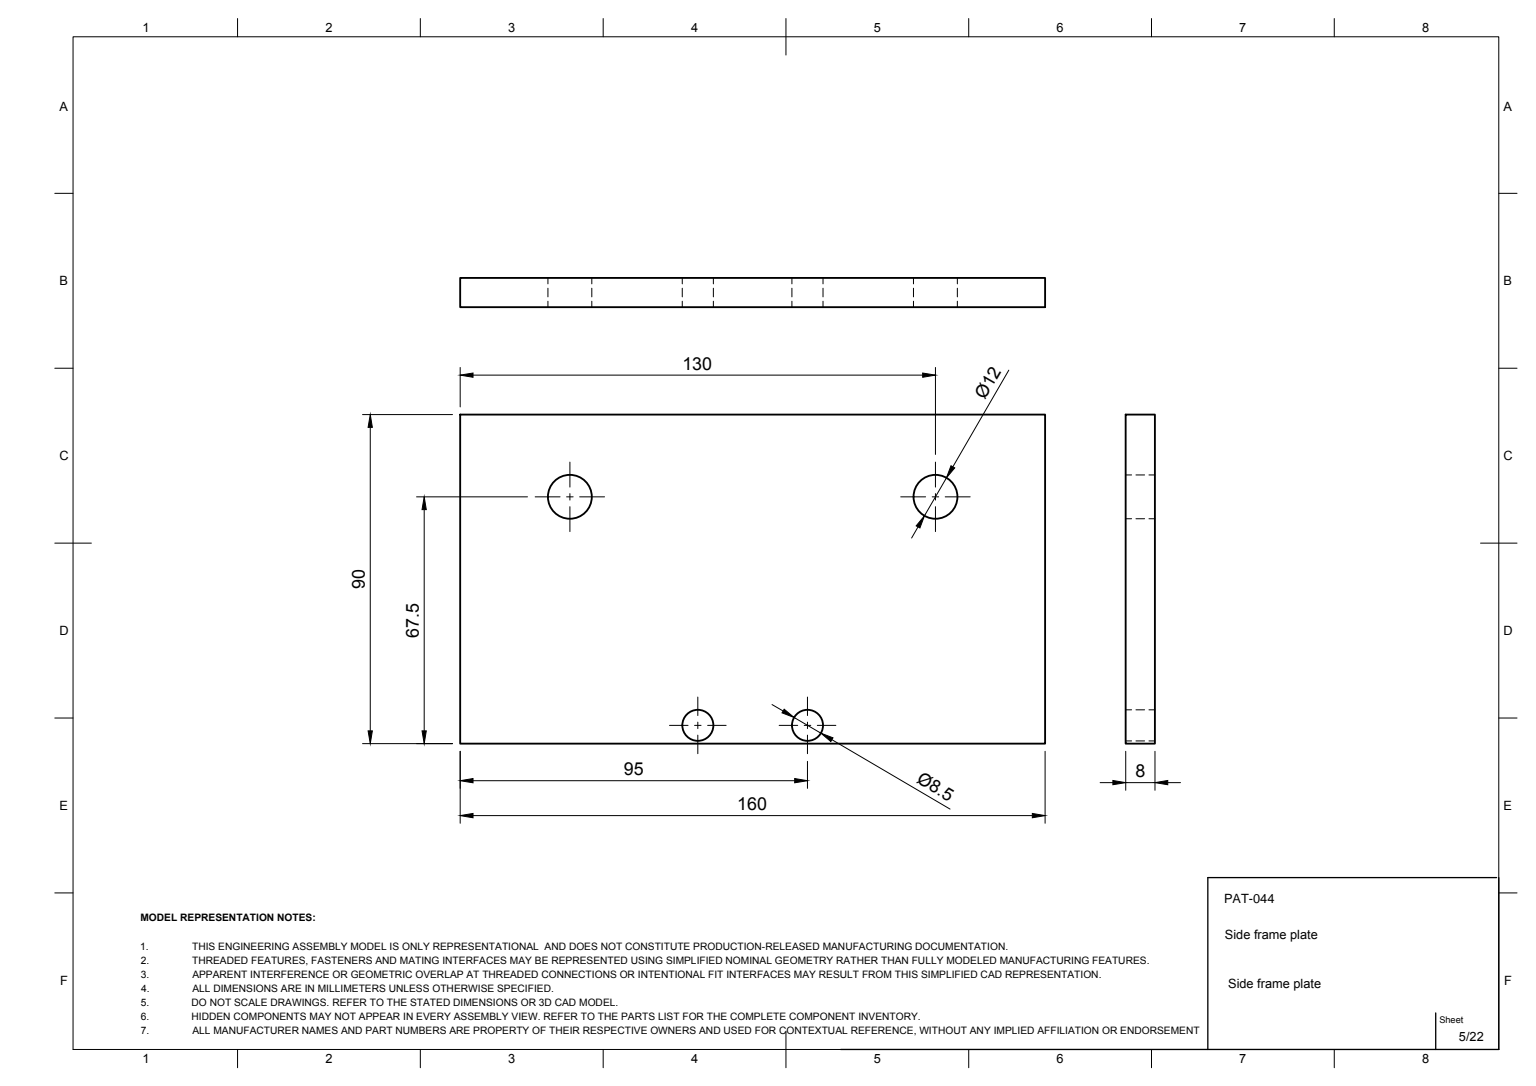
ISO-10303-21;
HEADER;
/* Generated by software containing ST-Developer
 * from STEP Tools, Inc. (www.steptools.com) 
 */

FILE_DESCRIPTION(
/* description */ ('Four-wheel beam trolley'),
/* implementation_level */ '2;1');

FILE_NAME(
/* name */ 'Side frame plate.step',
/* time_stamp */ '2026-10-29T16:22:06-07:00',
/* author */ (''),
/* organization */ (''),
/* preprocessor_version */ 'ST-DEVELOPER v20.2',
/* originating_system */ 'Autodesk Translation Framework v15.17.0.0',
/* authorisation */ '');

FILE_SCHEMA (('AUTOMOTIVE_DESIGN { 1 0 10303 214 3 1 1 }'));
ENDSEC;

DATA;
#10=MECHANICAL_DESIGN_GEOMETRIC_PRESENTATION_REPRESENTATION('',(#279),#4777);
#245=SHAPE_REPRESENTATION_RELATIONSHIP('SRR','None',#4874,#262);
#262=ADVANCED_BREP_SHAPE_REPRESENTATION('',(#303),#4759);
#279=STYLED_ITEM('',(#5035),#303);
#303=MANIFOLD_SOLID_BREP('Body1',#2366);
#328=FACE_BOUND('',#612,.T.);
#329=FACE_BOUND('',#613,.T.);
#330=FACE_BOUND('',#614,.T.);
#331=FACE_BOUND('',#615,.T.);
#332=FACE_BOUND('',#618,.T.);
#333=FACE_BOUND('',#619,.T.);
#334=FACE_BOUND('',#620,.T.);
#335=FACE_BOUND('',#621,.T.);
#375=PLANE('',#2617);
#376=PLANE('',#2618);
#377=PLANE('',#2619);
#378=PLANE('',#2620);
#379=PLANE('',#2621);
#380=PLANE('',#2622);
#456=FACE_OUTER_BOUND('',#607,.T.);
#457=FACE_OUTER_BOUND('',#608,.T.);
#458=FACE_OUTER_BOUND('',#609,.T.);
#459=FACE_OUTER_BOUND('',#610,.T.);
#460=FACE_OUTER_BOUND('',#611,.T.);
#461=FACE_OUTER_BOUND('',#616,.T.);
#462=FACE_OUTER_BOUND('',#617,.T.);
#463=FACE_OUTER_BOUND('',#622,.T.);
#464=FACE_OUTER_BOUND('',#623,.T.);
#465=FACE_OUTER_BOUND('',#624,.T.);
#607=EDGE_LOOP('',(#1673,#1674,#1675,#1676));
#608=EDGE_LOOP('',(#1677,#1678,#1679,#1680));
#609=EDGE_LOOP('',(#1681,#1682,#1683,#1684));
#610=EDGE_LOOP('',(#1685,#1686,#1687,#1688));
#611=EDGE_LOOP('',(#1689,#1690,#1691,#1692));
#612=EDGE_LOOP('',(#1693));
#613=EDGE_LOOP('',(#1694));
#614=EDGE_LOOP('',(#1695));
#615=EDGE_LOOP('',(#1696));
#616=EDGE_LOOP('',(#1697,#1698,#1699,#1700));
#617=EDGE_LOOP('',(#1701,#1702,#1703,#1704));
#618=EDGE_LOOP('',(#1705));
#619=EDGE_LOOP('',(#1706));
#620=EDGE_LOOP('',(#1707));
#621=EDGE_LOOP('',(#1708));
#622=EDGE_LOOP('',(#1709,#1710,#1711,#1712));
#623=EDGE_LOOP('',(#1713,#1714,#1715,#1716));
#624=EDGE_LOOP('',(#1717,#1718,#1719,#1720));
#793=LINE('',#3823,#916);
#794=LINE('',#3829,#917);
#795=LINE('',#3835,#918);
#796=LINE('',#3841,#919);
#797=LINE('',#3846,#920);
#798=LINE('',#3848,#921);
#799=LINE('',#3850,#922);
#800=LINE('',#3851,#923);
#801=LINE('',#3854,#924);
#802=LINE('',#3856,#925);
#803=LINE('',#3857,#926);
#804=LINE('',#3860,#927);
#805=LINE('',#3862,#928);
#806=LINE('',#3863,#929);
#807=LINE('',#3865,#930);
#808=LINE('',#3866,#931);
#916=VECTOR('',#3004,0.425);
#917=VECTOR('',#3011,0.425);
#918=VECTOR('',#3018,0.6);
#919=VECTOR('',#3025,0.6);
#920=VECTOR('',#3030,1.);
#921=VECTOR('',#3031,1.);
#922=VECTOR('',#3032,1.);
#923=VECTOR('',#3033,1.);
#924=VECTOR('',#3036,1.);
#925=VECTOR('',#3037,1.);
#926=VECTOR('',#3038,1.);
#927=VECTOR('',#3041,1.);
#928=VECTOR('',#3042,1.);
#929=VECTOR('',#3043,1.);
#930=VECTOR('',#3046,1.);
#931=VECTOR('',#3047,1.);
#1031=CIRCLE('',#2606,0.425);
#1032=CIRCLE('',#2607,0.425);
#1033=CIRCLE('',#2609,0.425);
#1034=CIRCLE('',#2610,0.425);
#1035=CIRCLE('',#2612,0.6);
#1036=CIRCLE('',#2613,0.6);
#1037=CIRCLE('',#2615,0.6);
#1038=CIRCLE('',#2616,0.6);
#1177=VERTEX_POINT('',#3820);
#1178=VERTEX_POINT('',#3822);
#1179=VERTEX_POINT('',#3826);
#1180=VERTEX_POINT('',#3828);
#1181=VERTEX_POINT('',#3832);
#1182=VERTEX_POINT('',#3834);
#1183=VERTEX_POINT('',#3838);
#1184=VERTEX_POINT('',#3840);
#1185=VERTEX_POINT('',#3844);
#1186=VERTEX_POINT('',#3845);
#1187=VERTEX_POINT('',#3847);
#1188=VERTEX_POINT('',#3849);
#1189=VERTEX_POINT('',#3853);
#1190=VERTEX_POINT('',#3855);
#1191=VERTEX_POINT('',#3859);
#1192=VERTEX_POINT('',#3861);
#1374=EDGE_CURVE('',#1177,#1177,#1031,.T.);
#1375=EDGE_CURVE('',#1177,#1178,#793,.T.);
#1376=EDGE_CURVE('',#1178,#1178,#1032,.T.);
#1377=EDGE_CURVE('',#1179,#1179,#1033,.T.);
#1378=EDGE_CURVE('',#1179,#1180,#794,.T.);
#1379=EDGE_CURVE('',#1180,#1180,#1034,.T.);
#1380=EDGE_CURVE('',#1181,#1181,#1035,.T.);
#1381=EDGE_CURVE('',#1181,#1182,#795,.T.);
#1382=EDGE_CURVE('',#1182,#1182,#1036,.T.);
#1383=EDGE_CURVE('',#1183,#1183,#1037,.T.);
#1384=EDGE_CURVE('',#1183,#1184,#796,.T.);
#1385=EDGE_CURVE('',#1184,#1184,#1038,.T.);
#1386=EDGE_CURVE('',#1185,#1186,#797,.T.);
#1387=EDGE_CURVE('',#1186,#1187,#798,.T.);
#1388=EDGE_CURVE('',#1188,#1187,#799,.T.);
#1389=EDGE_CURVE('',#1185,#1188,#800,.T.);
#1390=EDGE_CURVE('',#1189,#1185,#801,.T.);
#1391=EDGE_CURVE('',#1190,#1188,#802,.T.);
#1392=EDGE_CURVE('',#1189,#1190,#803,.T.);
#1393=EDGE_CURVE('',#1191,#1189,#804,.T.);
#1394=EDGE_CURVE('',#1192,#1190,#805,.T.);
#1395=EDGE_CURVE('',#1191,#1192,#806,.T.);
#1396=EDGE_CURVE('',#1186,#1191,#807,.T.);
#1397=EDGE_CURVE('',#1187,#1192,#808,.T.);
#1673=ORIENTED_EDGE('',*,*,#1374,.F.);
#1674=ORIENTED_EDGE('',*,*,#1375,.T.);
#1675=ORIENTED_EDGE('',*,*,#1376,.F.);
#1676=ORIENTED_EDGE('',*,*,#1375,.F.);
#1677=ORIENTED_EDGE('',*,*,#1377,.F.);
#1678=ORIENTED_EDGE('',*,*,#1378,.T.);
#1679=ORIENTED_EDGE('',*,*,#1379,.F.);
#1680=ORIENTED_EDGE('',*,*,#1378,.F.);
#1681=ORIENTED_EDGE('',*,*,#1380,.F.);
#1682=ORIENTED_EDGE('',*,*,#1381,.T.);
#1683=ORIENTED_EDGE('',*,*,#1382,.F.);
#1684=ORIENTED_EDGE('',*,*,#1381,.F.);
#1685=ORIENTED_EDGE('',*,*,#1383,.F.);
#1686=ORIENTED_EDGE('',*,*,#1384,.T.);
#1687=ORIENTED_EDGE('',*,*,#1385,.F.);
#1688=ORIENTED_EDGE('',*,*,#1384,.F.);
#1689=ORIENTED_EDGE('',*,*,#1386,.T.);
#1690=ORIENTED_EDGE('',*,*,#1387,.T.);
#1691=ORIENTED_EDGE('',*,*,#1388,.F.);
#1692=ORIENTED_EDGE('',*,*,#1389,.F.);
#1693=ORIENTED_EDGE('',*,*,#1376,.T.);
#1694=ORIENTED_EDGE('',*,*,#1379,.T.);
#1695=ORIENTED_EDGE('',*,*,#1382,.T.);
#1696=ORIENTED_EDGE('',*,*,#1385,.T.);
#1697=ORIENTED_EDGE('',*,*,#1390,.T.);
#1698=ORIENTED_EDGE('',*,*,#1389,.T.);
#1699=ORIENTED_EDGE('',*,*,#1391,.F.);
#1700=ORIENTED_EDGE('',*,*,#1392,.F.);
#1701=ORIENTED_EDGE('',*,*,#1393,.T.);
#1702=ORIENTED_EDGE('',*,*,#1392,.T.);
#1703=ORIENTED_EDGE('',*,*,#1394,.F.);
#1704=ORIENTED_EDGE('',*,*,#1395,.F.);
#1705=ORIENTED_EDGE('',*,*,#1374,.T.);
#1706=ORIENTED_EDGE('',*,*,#1377,.T.);
#1707=ORIENTED_EDGE('',*,*,#1380,.T.);
#1708=ORIENTED_EDGE('',*,*,#1383,.T.);
#1709=ORIENTED_EDGE('',*,*,#1396,.T.);
#1710=ORIENTED_EDGE('',*,*,#1395,.T.);
#1711=ORIENTED_EDGE('',*,*,#1397,.F.);
#1712=ORIENTED_EDGE('',*,*,#1387,.F.);
#1713=ORIENTED_EDGE('',*,*,#1397,.T.);
#1714=ORIENTED_EDGE('',*,*,#1394,.T.);
#1715=ORIENTED_EDGE('',*,*,#1391,.T.);
#1716=ORIENTED_EDGE('',*,*,#1388,.T.);
#1717=ORIENTED_EDGE('',*,*,#1396,.F.);
#1718=ORIENTED_EDGE('',*,*,#1386,.F.);
#1719=ORIENTED_EDGE('',*,*,#1390,.F.);
#1720=ORIENTED_EDGE('',*,*,#1393,.F.);
#2179=CYLINDRICAL_SURFACE('',#2605,0.425);
#2180=CYLINDRICAL_SURFACE('',#2608,0.425);
#2181=CYLINDRICAL_SURFACE('',#2611,0.6);
#2182=CYLINDRICAL_SURFACE('',#2614,0.6);
#2232=ADVANCED_FACE('',(#456),#2179,.F.);
#2233=ADVANCED_FACE('',(#457),#2180,.F.);
#2234=ADVANCED_FACE('',(#458),#2181,.F.);
#2235=ADVANCED_FACE('',(#459),#2182,.F.);
#2236=ADVANCED_FACE('',(#460,#328,#329,#330,#331),#375,.T.);
#2237=ADVANCED_FACE('',(#461),#376,.T.);
#2238=ADVANCED_FACE('',(#462,#332,#333,#334,#335),#377,.T.);
#2239=ADVANCED_FACE('',(#463),#378,.T.);
#2240=ADVANCED_FACE('',(#464),#379,.T.);
#2241=ADVANCED_FACE('',(#465),#380,.F.);
#2366=CLOSED_SHELL('',(#2232,#2233,#2234,#2235,#2236,#2237,#2238,#2239,
#2240,#2241));
#2604=AXIS2_PLACEMENT_3D('',#3818,#2998,#2999);
#2605=AXIS2_PLACEMENT_3D('',#3819,#3000,#3001);
#2606=AXIS2_PLACEMENT_3D('',#3821,#3002,#3003);
#2607=AXIS2_PLACEMENT_3D('',#3824,#3005,#3006);
#2608=AXIS2_PLACEMENT_3D('',#3825,#3007,#3008);
#2609=AXIS2_PLACEMENT_3D('',#3827,#3009,#3010);
#2610=AXIS2_PLACEMENT_3D('',#3830,#3012,#3013);
#2611=AXIS2_PLACEMENT_3D('',#3831,#3014,#3015);
#2612=AXIS2_PLACEMENT_3D('',#3833,#3016,#3017);
#2613=AXIS2_PLACEMENT_3D('',#3836,#3019,#3020);
#2614=AXIS2_PLACEMENT_3D('',#3837,#3021,#3022);
#2615=AXIS2_PLACEMENT_3D('',#3839,#3023,#3024);
#2616=AXIS2_PLACEMENT_3D('',#3842,#3026,#3027);
#2617=AXIS2_PLACEMENT_3D('',#3843,#3028,#3029);
#2618=AXIS2_PLACEMENT_3D('',#3852,#3034,#3035);
#2619=AXIS2_PLACEMENT_3D('',#3858,#3039,#3040);
#2620=AXIS2_PLACEMENT_3D('',#3864,#3044,#3045);
#2621=AXIS2_PLACEMENT_3D('',#3867,#3048,#3049);
#2622=AXIS2_PLACEMENT_3D('',#3868,#3050,#3051);
#2998=DIRECTION('axis',(0.,0.,1.));
#2999=DIRECTION('refdir',(1.,0.,0.));
#3000=DIRECTION('center_axis',(0.,1.,0.));
#3001=DIRECTION('ref_axis',(1.,0.,0.));
#3002=DIRECTION('center_axis',(0.,1.,0.));
#3003=DIRECTION('ref_axis',(1.,0.,0.));
#3004=DIRECTION('',(0.,1.,0.));
#3005=DIRECTION('center_axis',(0.,-1.,0.));
#3006=DIRECTION('ref_axis',(1.,0.,0.));
#3007=DIRECTION('center_axis',(0.,1.,0.));
#3008=DIRECTION('ref_axis',(1.,0.,0.));
#3009=DIRECTION('center_axis',(0.,1.,0.));
#3010=DIRECTION('ref_axis',(1.,0.,0.));
#3011=DIRECTION('',(0.,1.,0.));
#3012=DIRECTION('center_axis',(0.,-1.,0.));
#3013=DIRECTION('ref_axis',(1.,0.,0.));
#3014=DIRECTION('center_axis',(0.,1.,0.));
#3015=DIRECTION('ref_axis',(1.,0.,0.));
#3016=DIRECTION('center_axis',(0.,1.,0.));
#3017=DIRECTION('ref_axis',(1.,0.,0.));
#3018=DIRECTION('',(0.,1.,0.));
#3019=DIRECTION('center_axis',(0.,-1.,0.));
#3020=DIRECTION('ref_axis',(1.,0.,0.));
#3021=DIRECTION('center_axis',(0.,1.,0.));
#3022=DIRECTION('ref_axis',(1.,0.,0.));
#3023=DIRECTION('center_axis',(0.,1.,0.));
#3024=DIRECTION('ref_axis',(1.,0.,0.));
#3025=DIRECTION('',(0.,1.,0.));
#3026=DIRECTION('center_axis',(0.,-1.,0.));
#3027=DIRECTION('ref_axis',(1.,0.,0.));
#3028=DIRECTION('center_axis',(0.,1.,0.));
#3029=DIRECTION('ref_axis',(-1.,0.,0.));
#3030=DIRECTION('',(-1.,0.,0.));
#3031=DIRECTION('',(0.,0.,1.));
#3032=DIRECTION('',(-1.,0.,0.));
#3033=DIRECTION('',(0.,0.,1.));
#3034=DIRECTION('center_axis',(1.,0.,0.));
#3035=DIRECTION('ref_axis',(0.,1.,0.));
#3036=DIRECTION('',(0.,1.,0.));
#3037=DIRECTION('',(0.,1.,0.));
#3038=DIRECTION('',(0.,0.,1.));
#3039=DIRECTION('center_axis',(0.,-1.,0.));
#3040=DIRECTION('ref_axis',(1.,0.,0.));
#3041=DIRECTION('',(1.,0.,0.));
#3042=DIRECTION('',(1.,0.,0.));
#3043=DIRECTION('',(0.,0.,1.));
#3044=DIRECTION('center_axis',(-1.,0.,0.));
#3045=DIRECTION('ref_axis',(0.,-1.,0.));
#3046=DIRECTION('',(0.,-1.,0.));
#3047=DIRECTION('',(0.,-1.,0.));
#3048=DIRECTION('center_axis',(0.,0.,1.));
#3049=DIRECTION('ref_axis',(1.,0.,0.));
#3050=DIRECTION('center_axis',(0.,0.,1.));
#3051=DIRECTION('ref_axis',(1.,0.,0.));
#3818=CARTESIAN_POINT('',(0.,0.,0.));
#3819=CARTESIAN_POINT('Origin',(-1.5,5.4,7.5));
#3820=CARTESIAN_POINT('',(-1.925,5.5,7.5));
#3821=CARTESIAN_POINT('Origin',(-1.5,5.5,7.5));
#3822=CARTESIAN_POINT('',(-1.925,6.3,7.5));
#3823=CARTESIAN_POINT('',(-1.925,5.4,7.5));
#3824=CARTESIAN_POINT('Origin',(-1.5,6.3,7.5));
#3825=CARTESIAN_POINT('Origin',(1.5,5.4,7.5));
#3826=CARTESIAN_POINT('',(1.075,5.5,7.5));
#3827=CARTESIAN_POINT('Origin',(1.5,5.5,7.5));
#3828=CARTESIAN_POINT('',(1.075,6.3,7.5));
#3829=CARTESIAN_POINT('',(1.075,5.4,7.5));
#3830=CARTESIAN_POINT('Origin',(1.5,6.3,7.5));
#3831=CARTESIAN_POINT('Origin',(-5.,5.4,13.75));
#3832=CARTESIAN_POINT('',(-5.6,5.5,13.75));
#3833=CARTESIAN_POINT('Origin',(-5.,5.5,13.75));
#3834=CARTESIAN_POINT('',(-5.6,6.3,13.75));
#3835=CARTESIAN_POINT('',(-5.6,5.4,13.75));
#3836=CARTESIAN_POINT('Origin',(-5.,6.3,13.75));
#3837=CARTESIAN_POINT('Origin',(5.,5.4,13.75));
#3838=CARTESIAN_POINT('',(4.4,5.5,13.75));
#3839=CARTESIAN_POINT('Origin',(5.,5.5,13.75));
#3840=CARTESIAN_POINT('',(4.4,6.3,13.75));
#3841=CARTESIAN_POINT('',(4.4,5.4,13.75));
#3842=CARTESIAN_POINT('Origin',(5.,6.3,13.75));
#3843=CARTESIAN_POINT('Origin',(8.,6.3,7.));
#3844=CARTESIAN_POINT('',(8.,6.3,7.));
#3845=CARTESIAN_POINT('',(-8.,6.3,7.));
#3846=CARTESIAN_POINT('',(8.,6.3,7.));
#3847=CARTESIAN_POINT('',(-8.,6.3,16.));
#3848=CARTESIAN_POINT('',(-8.,6.3,7.));
#3849=CARTESIAN_POINT('',(8.,6.3,16.));
#3850=CARTESIAN_POINT('',(8.,6.3,16.));
#3851=CARTESIAN_POINT('',(8.,6.3,7.));
#3852=CARTESIAN_POINT('Origin',(8.,5.5,7.));
#3853=CARTESIAN_POINT('',(8.,5.5,7.));
#3854=CARTESIAN_POINT('',(8.,5.5,7.));
#3855=CARTESIAN_POINT('',(8.,5.5,16.));
#3856=CARTESIAN_POINT('',(8.,5.5,16.));
#3857=CARTESIAN_POINT('',(8.,5.5,7.));
#3858=CARTESIAN_POINT('Origin',(-8.,5.5,7.));
#3859=CARTESIAN_POINT('',(-8.,5.5,7.));
#3860=CARTESIAN_POINT('',(-8.,5.5,7.));
#3861=CARTESIAN_POINT('',(-8.,5.5,16.));
#3862=CARTESIAN_POINT('',(-8.,5.5,16.));
#3863=CARTESIAN_POINT('',(-8.,5.5,7.));
#3864=CARTESIAN_POINT('Origin',(-8.,6.3,7.));
#3865=CARTESIAN_POINT('',(-8.,6.3,7.));
#3866=CARTESIAN_POINT('',(-8.,6.3,16.));
#3867=CARTESIAN_POINT('Origin',(0.,5.9,16.));
#3868=CARTESIAN_POINT('Origin',(0.,5.9,7.));
#4737=UNCERTAINTY_MEASURE_WITH_UNIT(LENGTH_MEASURE(0.001),#4778,
'DISTANCE_ACCURACY_VALUE',
'Maximum model space distance between geometric entities at asserted c
onnectivities');
#4755=UNCERTAINTY_MEASURE_WITH_UNIT(LENGTH_MEASURE(0.001),#4778,
'DISTANCE_ACCURACY_VALUE',
'Maximum model space distance between geometric entities at asserted c
onnectivities');
#4759=(
GEOMETRIC_REPRESENTATION_CONTEXT(3)
GLOBAL_UNCERTAINTY_ASSIGNED_CONTEXT((#4737))
GLOBAL_UNIT_ASSIGNED_CONTEXT((#4778,#4780,#4781))
REPRESENTATION_CONTEXT('','3D')
);
#4777=(
GEOMETRIC_REPRESENTATION_CONTEXT(3)
GLOBAL_UNCERTAINTY_ASSIGNED_CONTEXT((#4755))
GLOBAL_UNIT_ASSIGNED_CONTEXT((#4778,#4780,#4781))
REPRESENTATION_CONTEXT('','3D')
);
#4778=(
LENGTH_UNIT()
NAMED_UNIT(*)
SI_UNIT(.CENTI.,.METRE.)
);
#4780=(
NAMED_UNIT(*)
PLANE_ANGLE_UNIT()
SI_UNIT($,.RADIAN.)
);
#4781=(
NAMED_UNIT(*)
SI_UNIT($,.STERADIAN.)
SOLID_ANGLE_UNIT()
);
#4785=SHAPE_DEFINITION_REPRESENTATION(#4806,#4874);
#4806=PRODUCT_DEFINITION_SHAPE('',$,#4896);
#4874=SHAPE_REPRESENTATION('',(#2604),#4759);
#4892=PRODUCT_DEFINITION_CONTEXT('part definition',#4957,'design');
#4896=PRODUCT_DEFINITION('Side frame plate','Side frame plate',#4917,#4892);
#4917=PRODUCT_DEFINITION_FORMATION('',$,#4962);
#4957=APPLICATION_CONTEXT(
'Core Data for Automotive Mechanical Design Process');
#4958=PRODUCT_CONTEXT('part definition',#4957,'mechanical');
#4962=PRODUCT('Side frame plate','Side frame plate','Side frame plate',
(#4958));
#5029=COLOUR_RGB('Dark Blue',0.08,0.2,0.34);
#5030=FILL_AREA_STYLE_COLOUR('',#5029);
#5031=FILL_AREA_STYLE('',(#5030));
#5032=SURFACE_STYLE_FILL_AREA(#5031);
#5033=SURFACE_SIDE_STYLE('',(#5032));
#5034=SURFACE_STYLE_USAGE(.BOTH.,#5033);
#5035=PRESENTATION_STYLE_ASSIGNMENT((#5034));
ENDSEC;
END-ISO-10303-21;
